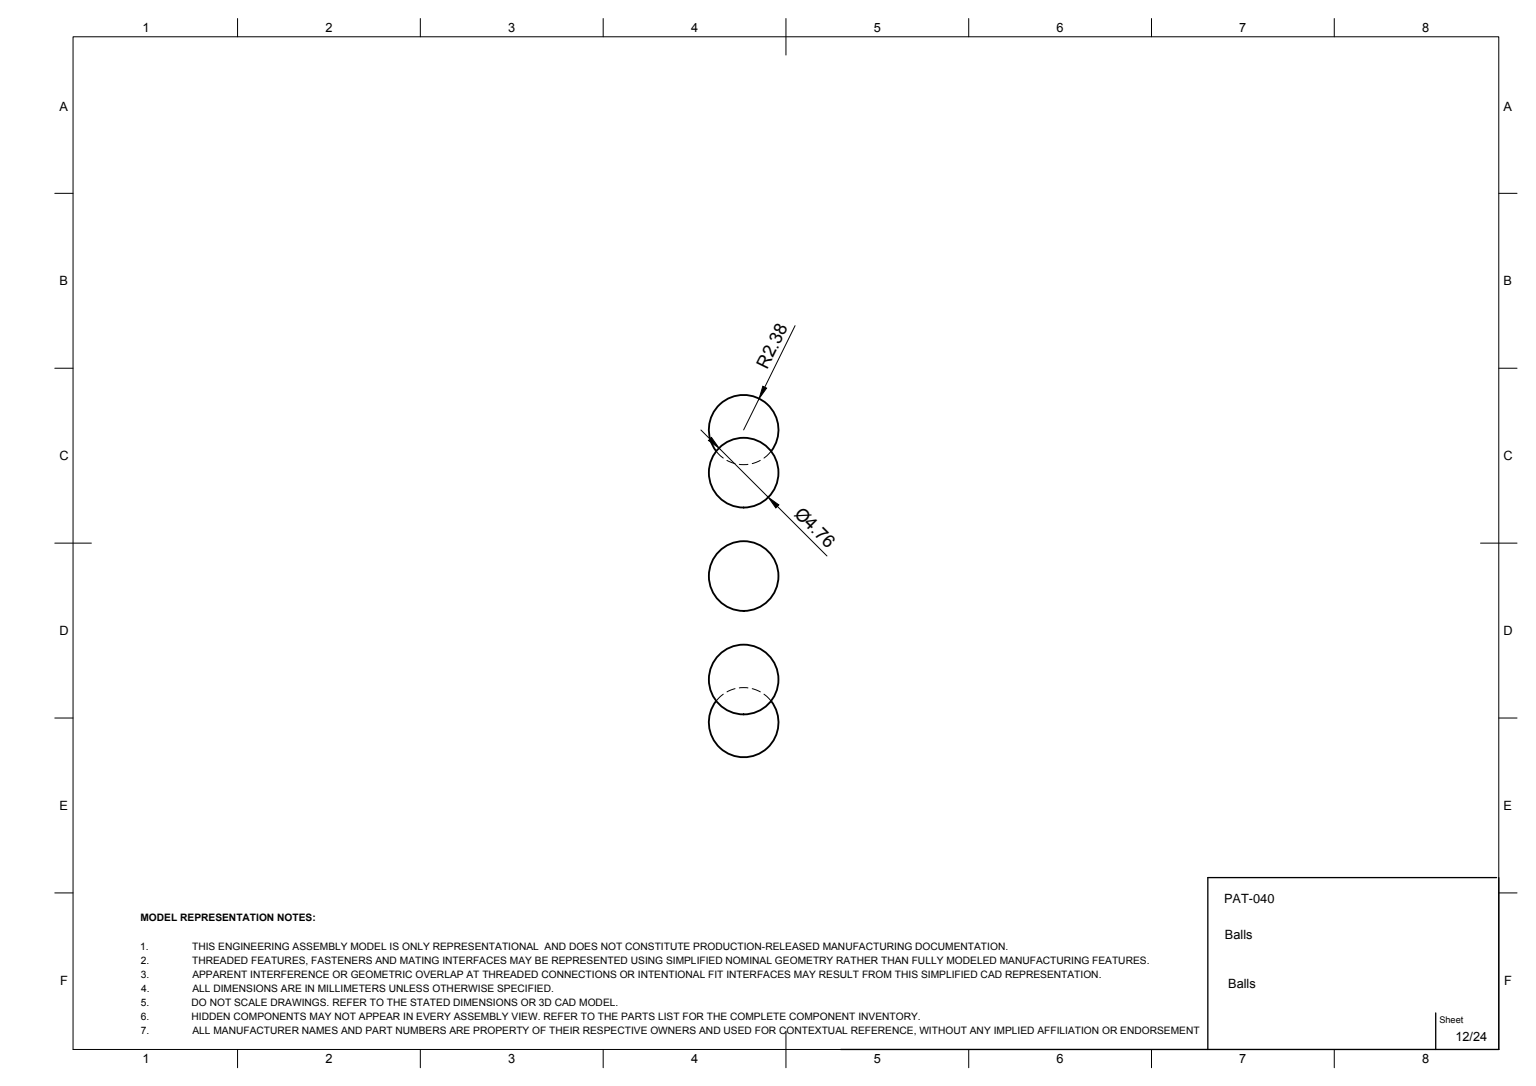
ISO-10303-21;
HEADER;
/* Generated by software containing ST-Developer
 * from STEP Tools, Inc. (www.steptools.com) 
 */

FILE_DESCRIPTION(
/* description */ ('Four-bar tabletop demonstrator'),
/* implementation_level */ '2;1');

FILE_NAME(
/* name */ 'Balls.step',
/* time_stamp */ '2026-10-29T17:05:23-07:00',
/* author */ (''),
/* organization */ (''),
/* preprocessor_version */ 'ST-DEVELOPER v20.2',
/* originating_system */ 'Autodesk Translation Framework v15.17.0.0',
/* authorisation */ '');

FILE_SCHEMA (('AUTOMOTIVE_DESIGN { 1 0 10303 214 3 1 1 }'));
ENDSEC;

DATA;
#10=MECHANICAL_DESIGN_GEOMETRIC_PRESENTATION_REPRESENTATION('',(#343,#344,#345,#346,#347,#348,#349,#350),#6705);
#247=SPHERICAL_SURFACE('',#3789,0.23815);
#248=SPHERICAL_SURFACE('',#3791,0.23815);
#249=SPHERICAL_SURFACE('',#3793,0.23815);
#250=SPHERICAL_SURFACE('',#3795,0.23815);
#251=SPHERICAL_SURFACE('',#3797,0.23815);
#252=SPHERICAL_SURFACE('',#3799,0.23815);
#253=SPHERICAL_SURFACE('',#3801,0.23815);
#254=SPHERICAL_SURFACE('',#3803,0.23815);
#313=SHAPE_REPRESENTATION_RELATIONSHIP('SRR','None',#6822,#328);
#328=ADVANCED_BREP_SHAPE_REPRESENTATION('',(#365,#366,#367,#368,#369,#370,
#371,#372),#6695);
#343=STYLED_ITEM('',(#6989),#365);
#344=STYLED_ITEM('',(#6989),#366);
#345=STYLED_ITEM('',(#6989),#367);
#346=STYLED_ITEM('',(#6989),#368);
#347=STYLED_ITEM('',(#6989),#369);
#348=STYLED_ITEM('',(#6989),#370);
#349=STYLED_ITEM('',(#6989),#371);
#350=STYLED_ITEM('',(#6989),#372);
#365=MANIFOLD_SOLID_BREP('Body1',#3388);
#366=MANIFOLD_SOLID_BREP('Body2',#3389);
#367=MANIFOLD_SOLID_BREP('Body3',#3390);
#368=MANIFOLD_SOLID_BREP('Body4',#3391);
#369=MANIFOLD_SOLID_BREP('Body5',#3392);
#370=MANIFOLD_SOLID_BREP('Body6',#3393);
#371=MANIFOLD_SOLID_BREP('Body7',#3394);
#372=MANIFOLD_SOLID_BREP('Body8',#3395);
#660=FACE_OUTER_BOUND('',#912,.T.);
#661=FACE_OUTER_BOUND('',#913,.T.);
#662=FACE_OUTER_BOUND('',#914,.T.);
#663=FACE_OUTER_BOUND('',#915,.T.);
#664=FACE_OUTER_BOUND('',#916,.T.);
#665=FACE_OUTER_BOUND('',#917,.T.);
#666=FACE_OUTER_BOUND('',#918,.T.);
#667=FACE_OUTER_BOUND('',#919,.T.);
#912=EDGE_LOOP('',(#2692,#2693));
#913=EDGE_LOOP('',(#2694,#2695));
#914=EDGE_LOOP('',(#2696,#2697));
#915=EDGE_LOOP('',(#2698,#2699));
#916=EDGE_LOOP('',(#2700,#2701));
#917=EDGE_LOOP('',(#2702,#2703));
#918=EDGE_LOOP('',(#2704,#2705));
#919=EDGE_LOOP('',(#2706,#2707));
#1496=CIRCLE('',#3790,0.23815);
#1497=CIRCLE('',#3792,0.23815);
#1498=CIRCLE('',#3794,0.23815);
#1499=CIRCLE('',#3796,0.23815);
#1500=CIRCLE('',#3798,0.23815);
#1501=CIRCLE('',#3800,0.23815);
#1502=CIRCLE('',#3802,0.23815);
#1503=CIRCLE('',#3804,0.23815);
#1733=VERTEX_POINT('',#5738);
#1734=VERTEX_POINT('',#5739);
#1735=VERTEX_POINT('',#5742);
#1736=VERTEX_POINT('',#5743);
#1737=VERTEX_POINT('',#5746);
#1738=VERTEX_POINT('',#5747);
#1739=VERTEX_POINT('',#5750);
#1740=VERTEX_POINT('',#5751);
#1741=VERTEX_POINT('',#5754);
#1742=VERTEX_POINT('',#5755);
#1743=VERTEX_POINT('',#5758);
#1744=VERTEX_POINT('',#5759);
#1745=VERTEX_POINT('',#5762);
#1746=VERTEX_POINT('',#5763);
#1747=VERTEX_POINT('',#5766);
#1748=VERTEX_POINT('',#5767);
#2082=EDGE_CURVE('',#1733,#1734,#1496,.T.);
#2083=EDGE_CURVE('',#1735,#1736,#1497,.T.);
#2084=EDGE_CURVE('',#1737,#1738,#1498,.T.);
#2085=EDGE_CURVE('',#1739,#1740,#1499,.T.);
#2086=EDGE_CURVE('',#1741,#1742,#1500,.T.);
#2087=EDGE_CURVE('',#1743,#1744,#1501,.T.);
#2088=EDGE_CURVE('',#1745,#1746,#1502,.T.);
#2089=EDGE_CURVE('',#1747,#1748,#1503,.T.);
#2692=ORIENTED_EDGE('',*,*,#2082,.T.);
#2693=ORIENTED_EDGE('',*,*,#2082,.F.);
#2694=ORIENTED_EDGE('',*,*,#2083,.T.);
#2695=ORIENTED_EDGE('',*,*,#2083,.F.);
#2696=ORIENTED_EDGE('',*,*,#2084,.T.);
#2697=ORIENTED_EDGE('',*,*,#2084,.F.);
#2698=ORIENTED_EDGE('',*,*,#2085,.T.);
#2699=ORIENTED_EDGE('',*,*,#2085,.F.);
#2700=ORIENTED_EDGE('',*,*,#2086,.T.);
#2701=ORIENTED_EDGE('',*,*,#2086,.F.);
#2702=ORIENTED_EDGE('',*,*,#2087,.T.);
#2703=ORIENTED_EDGE('',*,*,#2087,.F.);
#2704=ORIENTED_EDGE('',*,*,#2088,.T.);
#2705=ORIENTED_EDGE('',*,*,#2088,.F.);
#2706=ORIENTED_EDGE('',*,*,#2089,.T.);
#2707=ORIENTED_EDGE('',*,*,#2089,.F.);
#3276=ADVANCED_FACE('',(#660),#247,.T.);
#3277=ADVANCED_FACE('',(#661),#248,.T.);
#3278=ADVANCED_FACE('',(#662),#249,.T.);
#3279=ADVANCED_FACE('',(#663),#250,.T.);
#3280=ADVANCED_FACE('',(#664),#251,.T.);
#3281=ADVANCED_FACE('',(#665),#252,.T.);
#3282=ADVANCED_FACE('',(#666),#253,.T.);
#3283=ADVANCED_FACE('',(#667),#254,.T.);
#3388=CLOSED_SHELL('',(#3276));
#3389=CLOSED_SHELL('',(#3277));
#3390=CLOSED_SHELL('',(#3278));
#3391=CLOSED_SHELL('',(#3279));
#3392=CLOSED_SHELL('',(#3280));
#3393=CLOSED_SHELL('',(#3281));
#3394=CLOSED_SHELL('',(#3282));
#3395=CLOSED_SHELL('',(#3283));
#3788=AXIS2_PLACEMENT_3D('',#5736,#4589,#4590);
#3789=AXIS2_PLACEMENT_3D('',#5737,#4591,#4592);
#3790=AXIS2_PLACEMENT_3D('',#5740,#4593,#4594);
#3791=AXIS2_PLACEMENT_3D('',#5741,#4595,#4596);
#3792=AXIS2_PLACEMENT_3D('',#5744,#4597,#4598);
#3793=AXIS2_PLACEMENT_3D('',#5745,#4599,#4600);
#3794=AXIS2_PLACEMENT_3D('',#5748,#4601,#4602);
#3795=AXIS2_PLACEMENT_3D('',#5749,#4603,#4604);
#3796=AXIS2_PLACEMENT_3D('',#5752,#4605,#4606);
#3797=AXIS2_PLACEMENT_3D('',#5753,#4607,#4608);
#3798=AXIS2_PLACEMENT_3D('',#5756,#4609,#4610);
#3799=AXIS2_PLACEMENT_3D('',#5757,#4611,#4612);
#3800=AXIS2_PLACEMENT_3D('',#5760,#4613,#4614);
#3801=AXIS2_PLACEMENT_3D('',#5761,#4615,#4616);
#3802=AXIS2_PLACEMENT_3D('',#5764,#4617,#4618);
#3803=AXIS2_PLACEMENT_3D('',#5765,#4619,#4620);
#3804=AXIS2_PLACEMENT_3D('',#5768,#4621,#4622);
#4589=DIRECTION('axis',(0.,0.,1.));
#4590=DIRECTION('refdir',(1.,0.,0.));
#4591=DIRECTION('center_axis',(0.,0.,1.));
#4592=DIRECTION('ref_axis',(1.,0.,0.));
#4593=DIRECTION('center_axis',(1.22464679914735E-16,-1.,0.));
#4594=DIRECTION('ref_axis',(-1.,-1.22464679914735E-16,0.));
#4595=DIRECTION('center_axis',(0.707106781186548,0.,0.707106781186548));
#4596=DIRECTION('ref_axis',(0.707106781186548,0.,-0.707106781186548));
#4597=DIRECTION('center_axis',(8.65956056235494E-17,-1.,-8.65956056235493E-17));
#4598=DIRECTION('ref_axis',(-0.707106781186547,-1.22464679914735E-16,0.707106781186547));
#4599=DIRECTION('center_axis',(1.,0.,0.));
#4600=DIRECTION('ref_axis',(6.12323399573676E-17,0.,-1.));
#4601=DIRECTION('center_axis',(7.49879891330929E-33,-1.,-1.22464679914735E-16));
#4602=DIRECTION('ref_axis',(-6.12323399573676E-17,-1.22464679914735E-16,
1.));
#4603=DIRECTION('center_axis',(0.707106781186548,0.,-0.707106781186548));
#4604=DIRECTION('ref_axis',(-0.707106781186548,0.,-0.707106781186548));
#4605=DIRECTION('center_axis',(-8.65956056235493E-17,-1.,-8.65956056235494E-17));
#4606=DIRECTION('ref_axis',(0.707106781186547,-1.22464679914735E-16,0.707106781186547));
#4607=DIRECTION('center_axis',(0.,0.,-1.));
#4608=DIRECTION('ref_axis',(-1.,0.,-1.22464679914735E-16));
#4609=DIRECTION('center_axis',(-1.22464679914735E-16,-1.,-1.49975978266186E-32));
#4610=DIRECTION('ref_axis',(1.,-1.22464679914735E-16,1.22464679914735E-16));
#4611=DIRECTION('center_axis',(-0.707106781186547,0.,-0.707106781186548));
#4612=DIRECTION('ref_axis',(-0.707106781186548,0.,0.707106781186547));
#4613=DIRECTION('center_axis',(-8.65956056235493E-17,-1.,8.65956056235493E-17));
#4614=DIRECTION('ref_axis',(0.707106781186548,-1.22464679914735E-16,-0.707106781186547));
#4615=DIRECTION('center_axis',(-1.,0.,0.));
#4616=DIRECTION('ref_axis',(-1.83697019872103E-16,0.,1.));
#4617=DIRECTION('center_axis',(-2.24963967399279E-32,-1.,1.22464679914735E-16));
#4618=DIRECTION('ref_axis',(1.83697019872103E-16,-1.22464679914735E-16,
-1.));
#4619=DIRECTION('center_axis',(-0.707106781186548,0.,0.707106781186548));
#4620=DIRECTION('ref_axis',(0.707106781186547,0.,0.707106781186548));
#4621=DIRECTION('center_axis',(8.65956056235493E-17,-1.,8.65956056235493E-17));
#4622=DIRECTION('ref_axis',(-0.707106781186547,-1.22464679914735E-16,-0.707106781186548));
#5736=CARTESIAN_POINT('',(0.,0.,0.));
#5737=CARTESIAN_POINT('Origin',(1.,0.,0.));
#5738=CARTESIAN_POINT('',(1.,-1.78583896120461E-33,0.23815));
#5739=CARTESIAN_POINT('',(1.,-1.78583896120461E-33,-0.23815));
#5740=CARTESIAN_POINT('Origin',(1.,0.,0.));
#5741=CARTESIAN_POINT('Origin',(0.707106781186548,0.,-0.707106781186547));
#5742=CARTESIAN_POINT('',(0.875504261126124,-1.78583896120461E-33,-0.538709301246971));
#5743=CARTESIAN_POINT('',(0.538709301246971,-1.78583896120461E-33,-0.875504261126124));
#5744=CARTESIAN_POINT('Origin',(0.707106781186548,0.,-0.707106781186547));
#5745=CARTESIAN_POINT('Origin',(6.12323399573677E-17,0.,-1.));
#5746=CARTESIAN_POINT('',(0.23815,-1.78583896120461E-33,-1.));
#5747=CARTESIAN_POINT('',(-0.23815,-1.78583896120461E-33,-1.));
#5748=CARTESIAN_POINT('Origin',(6.12323399573677E-17,0.,-1.));
#5749=CARTESIAN_POINT('Origin',(-0.707106781186547,0.,-0.707106781186548));
#5750=CARTESIAN_POINT('',(-0.538709301246971,-1.78583896120461E-33,-0.875504261126124));
#5751=CARTESIAN_POINT('',(-0.875504261126124,-1.78583896120461E-33,-0.538709301246971));
#5752=CARTESIAN_POINT('Origin',(-0.707106781186547,0.,-0.707106781186548));
#5753=CARTESIAN_POINT('Origin',(-1.,0.,-1.22464679914735E-16));
#5754=CARTESIAN_POINT('',(-1.,-1.78583896120461E-33,-0.23815));
#5755=CARTESIAN_POINT('',(-1.,-1.78583896120461E-33,0.23815));
#5756=CARTESIAN_POINT('Origin',(-1.,0.,-1.22464679914735E-16));
#5757=CARTESIAN_POINT('Origin',(-0.707106781186548,0.,0.707106781186547));
#5758=CARTESIAN_POINT('',(-0.875504261126124,-7.94881478324376E-33,0.538709301246971));
#5759=CARTESIAN_POINT('',(-0.538709301246971,4.37713686083455E-33,0.875504261126124));
#5760=CARTESIAN_POINT('Origin',(-0.707106781186548,0.,0.707106781186547));
#5761=CARTESIAN_POINT('Origin',(-1.83697019872103E-16,0.,1.));
#5762=CARTESIAN_POINT('',(-0.23815,-1.78583896120461E-33,1.));
#5763=CARTESIAN_POINT('',(0.23815,-1.78583896120461E-33,1.));
#5764=CARTESIAN_POINT('Origin',(-1.83697019872103E-16,0.,1.));
#5765=CARTESIAN_POINT('Origin',(0.707106781186547,0.,0.707106781186548));
#5766=CARTESIAN_POINT('',(0.538709301246971,-4.86732687222419E-33,0.875504261126124));
#5767=CARTESIAN_POINT('',(0.875504261126124,1.29564894981497E-33,0.538709301246971));
#5768=CARTESIAN_POINT('Origin',(0.707106781186547,0.,0.707106781186548));
#6673=UNCERTAINTY_MEASURE_WITH_UNIT(LENGTH_MEASURE(0.001),#6706,
'DISTANCE_ACCURACY_VALUE',
'Maximum model space distance between geometric entities at asserted c
onnectivities');
#6683=UNCERTAINTY_MEASURE_WITH_UNIT(LENGTH_MEASURE(0.001),#6706,
'DISTANCE_ACCURACY_VALUE',
'Maximum model space distance between geometric entities at asserted c
onnectivities');
#6695=(
GEOMETRIC_REPRESENTATION_CONTEXT(3)
GLOBAL_UNCERTAINTY_ASSIGNED_CONTEXT((#6673))
GLOBAL_UNIT_ASSIGNED_CONTEXT((#6706,#6708,#6709))
REPRESENTATION_CONTEXT('','3D')
);
#6705=(
GEOMETRIC_REPRESENTATION_CONTEXT(3)
GLOBAL_UNCERTAINTY_ASSIGNED_CONTEXT((#6683))
GLOBAL_UNIT_ASSIGNED_CONTEXT((#6706,#6708,#6709))
REPRESENTATION_CONTEXT('','3D')
);
#6706=(
LENGTH_UNIT()
NAMED_UNIT(*)
SI_UNIT(.CENTI.,.METRE.)
);
#6708=(
NAMED_UNIT(*)
PLANE_ANGLE_UNIT()
SI_UNIT($,.RADIAN.)
);
#6709=(
NAMED_UNIT(*)
SI_UNIT($,.STERADIAN.)
SOLID_ANGLE_UNIT()
);
#6721=SHAPE_DEFINITION_REPRESENTATION(#6742,#6822);
#6742=PRODUCT_DEFINITION_SHAPE('',$,#6844);
#6822=SHAPE_REPRESENTATION('',(#3788),#6695);
#6832=PRODUCT_DEFINITION_CONTEXT('part definition',#6897,'design');
#6844=PRODUCT_DEFINITION('Balls','Balls',#6865,#6832);
#6865=PRODUCT_DEFINITION_FORMATION('',$,#6910);
#6897=APPLICATION_CONTEXT(
'Core Data for Automotive Mechanical Design Process');
#6898=PRODUCT_CONTEXT('part definition',#6897,'mechanical');
#6910=PRODUCT('Balls','Balls','Balls',(#6898));
#6983=COLOUR_RGB('Grey',0.48,0.52,0.57);
#6984=FILL_AREA_STYLE_COLOUR('',#6983);
#6985=FILL_AREA_STYLE('',(#6984));
#6986=SURFACE_STYLE_FILL_AREA(#6985);
#6987=SURFACE_SIDE_STYLE('',(#6986));
#6988=SURFACE_STYLE_USAGE(.BOTH.,#6987);
#6989=PRESENTATION_STYLE_ASSIGNMENT((#6988));
ENDSEC;
END-ISO-10303-21;
